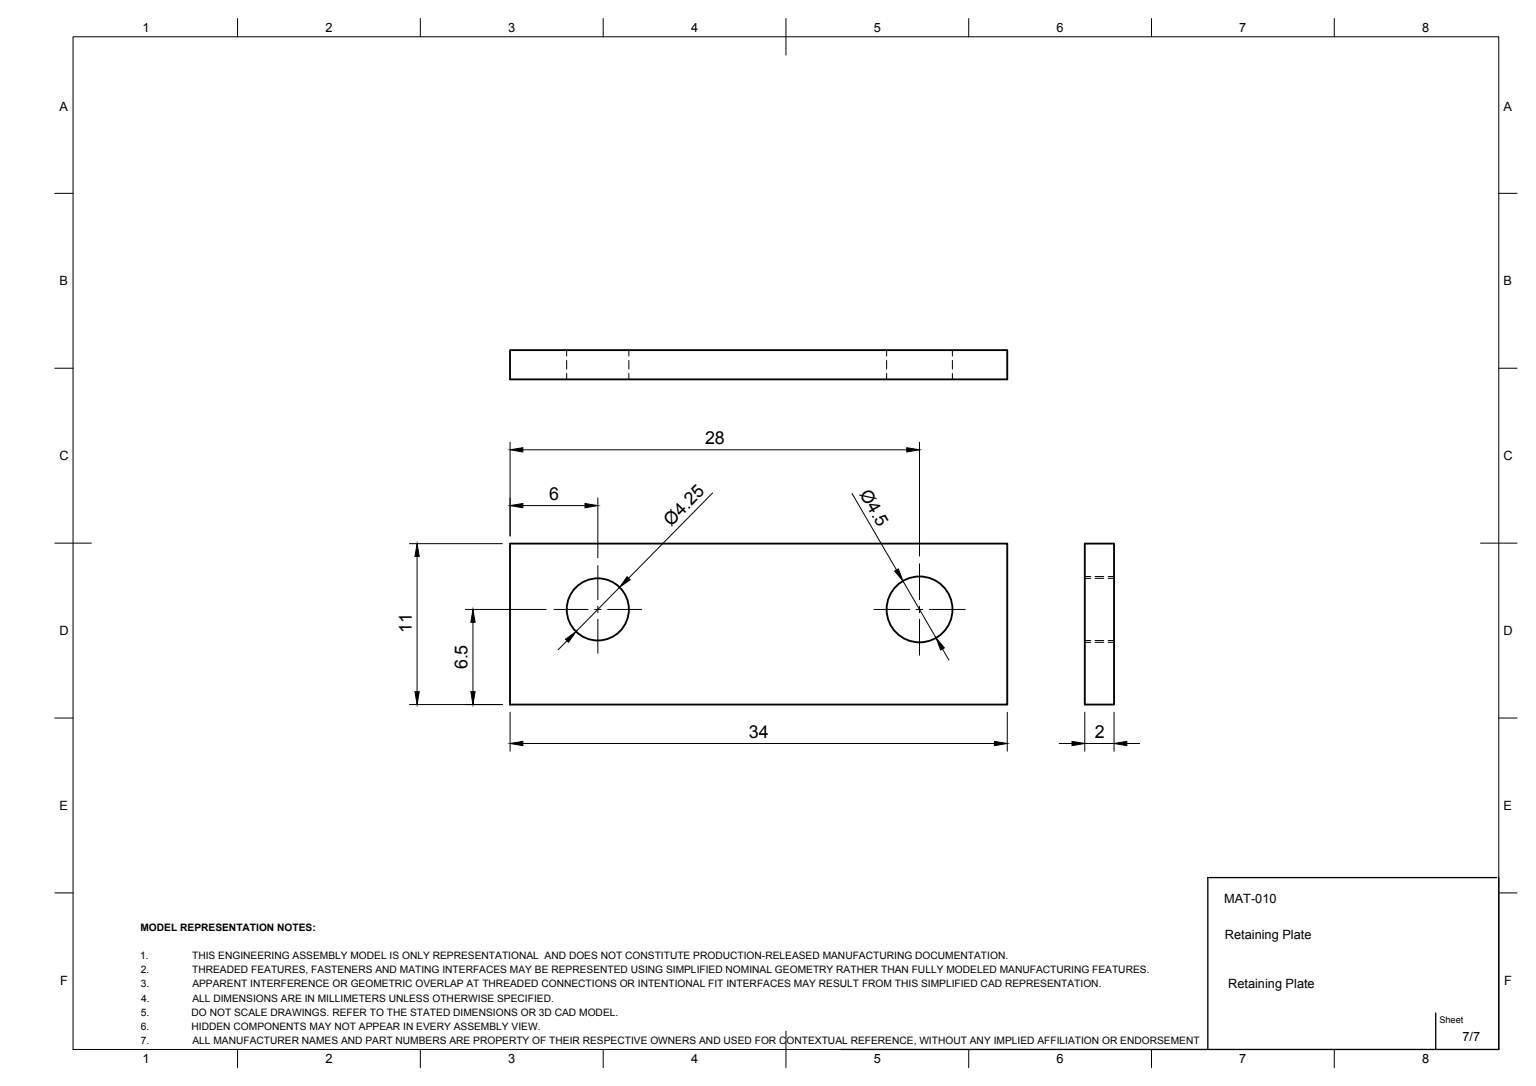
ISO-10303-21;
HEADER;
/* Generated by software containing ST-Developer
 * from STEP Tools, Inc. (www.steptools.com) 
 */

FILE_DESCRIPTION(
/* description */ ('STEP AP214'),
/* implementation_level */ '2;1');

FILE_NAME(
/* name */ 'Retaining Plate.step',
/* time_stamp */ '2026-11-14T05:50:49-08:00',
/* author */ (''),
/* organization */ (''),
/* preprocessor_version */ 'ST-DEVELOPER v20.2',
/* originating_system */ 'Autodesk Translation Framework v15.17.0.0',
/* authorisation */ '');

FILE_SCHEMA (('AUTOMOTIVE_DESIGN { 1 0 10303 214 3 1 1 }'));
ENDSEC;

DATA;
#10=MECHANICAL_DESIGN_GEOMETRIC_PRESENTATION_REPRESENTATION('',(#162),#9903);
#148=SHAPE_REPRESENTATION_RELATIONSHIP('SRR','None',#9943,#155);
#155=ADVANCED_BREP_SHAPE_REPRESENTATION('',(#169),#9901);
#162=STYLED_ITEM('',(#9984),#169);
#169=MANIFOLD_SOLID_BREP('Body1',#2027);
#191=FACE_BOUND('',#446,.T.);
#192=FACE_BOUND('',#447,.T.);
#193=FACE_BOUND('',#449,.T.);
#194=FACE_BOUND('',#450,.T.);
#224=PLANE('',#2228);
#225=PLANE('',#2229);
#226=PLANE('',#2230);
#227=PLANE('',#2231);
#228=PLANE('',#2232);
#229=PLANE('',#2233);
#305=FACE_OUTER_BOUND('',#443,.T.);
#306=FACE_OUTER_BOUND('',#444,.T.);
#307=FACE_OUTER_BOUND('',#445,.T.);
#308=FACE_OUTER_BOUND('',#448,.T.);
#309=FACE_OUTER_BOUND('',#451,.T.);
#310=FACE_OUTER_BOUND('',#452,.T.);
#311=FACE_OUTER_BOUND('',#453,.T.);
#312=FACE_OUTER_BOUND('',#454,.T.);
#443=EDGE_LOOP('',(#1520,#1521,#1522,#1523));
#444=EDGE_LOOP('',(#1524,#1525,#1526,#1527));
#445=EDGE_LOOP('',(#1528,#1529,#1530,#1531));
#446=EDGE_LOOP('',(#1532));
#447=EDGE_LOOP('',(#1533));
#448=EDGE_LOOP('',(#1534,#1535,#1536,#1537));
#449=EDGE_LOOP('',(#1538));
#450=EDGE_LOOP('',(#1539));
#451=EDGE_LOOP('',(#1540,#1541,#1542,#1543));
#452=EDGE_LOOP('',(#1544,#1545,#1546,#1547));
#453=EDGE_LOOP('',(#1548,#1549,#1550,#1551));
#454=EDGE_LOOP('',(#1552,#1553,#1554,#1555));
#563=LINE('',#3113,#699);
#564=LINE('',#3119,#700);
#565=LINE('',#3124,#701);
#566=LINE('',#3126,#702);
#567=LINE('',#3128,#703);
#568=LINE('',#3129,#704);
#569=LINE('',#3133,#705);
#570=LINE('',#3135,#706);
#571=LINE('',#3137,#707);
#572=LINE('',#3138,#708);
#573=LINE('',#3140,#709);
#574=LINE('',#3141,#710);
#575=LINE('',#3143,#711);
#576=LINE('',#3145,#712);
#699=VECTOR('',#2602,2.125);
#700=VECTOR('',#2609,2.25);
#701=VECTOR('',#2614,1000.);
#702=VECTOR('',#2615,1000.);
#703=VECTOR('',#2616,1000.);
#704=VECTOR('',#2617,1000.);
#705=VECTOR('',#2620,1000.);
#706=VECTOR('',#2621,1000.);
#707=VECTOR('',#2622,1000.);
#708=VECTOR('',#2623,1000.);
#709=VECTOR('',#2626,1000.);
#710=VECTOR('',#2627,1000.);
#711=VECTOR('',#2630,1000.);
#712=VECTOR('',#2633,1000.);
#840=CIRCLE('',#2223,2.125);
#841=CIRCLE('',#2224,2.125);
#842=CIRCLE('',#2226,2.25);
#843=CIRCLE('',#2227,2.25);
#927=VERTEX_POINT('',#3110);
#928=VERTEX_POINT('',#3112);
#929=VERTEX_POINT('',#3116);
#930=VERTEX_POINT('',#3118);
#931=VERTEX_POINT('',#3122);
#932=VERTEX_POINT('',#3123);
#933=VERTEX_POINT('',#3125);
#934=VERTEX_POINT('',#3127);
#935=VERTEX_POINT('',#3131);
#936=VERTEX_POINT('',#3132);
#937=VERTEX_POINT('',#3134);
#938=VERTEX_POINT('',#3136);
#1141=EDGE_CURVE('',#927,#927,#840,.T.);
#1142=EDGE_CURVE('',#927,#928,#563,.T.);
#1143=EDGE_CURVE('',#928,#928,#841,.T.);
#1144=EDGE_CURVE('',#929,#929,#842,.T.);
#1145=EDGE_CURVE('',#929,#930,#564,.T.);
#1146=EDGE_CURVE('',#930,#930,#843,.T.);
#1147=EDGE_CURVE('',#931,#932,#565,.T.);
#1148=EDGE_CURVE('',#932,#933,#566,.T.);
#1149=EDGE_CURVE('',#933,#934,#567,.T.);
#1150=EDGE_CURVE('',#934,#931,#568,.T.);
#1151=EDGE_CURVE('',#935,#936,#569,.T.);
#1152=EDGE_CURVE('',#937,#935,#570,.T.);
#1153=EDGE_CURVE('',#938,#937,#571,.T.);
#1154=EDGE_CURVE('',#936,#938,#572,.T.);
#1155=EDGE_CURVE('',#932,#936,#573,.T.);
#1156=EDGE_CURVE('',#931,#935,#574,.T.);
#1157=EDGE_CURVE('',#933,#938,#575,.T.);
#1158=EDGE_CURVE('',#934,#937,#576,.T.);
#1520=ORIENTED_EDGE('',*,*,#1141,.T.);
#1521=ORIENTED_EDGE('',*,*,#1142,.T.);
#1522=ORIENTED_EDGE('',*,*,#1143,.F.);
#1523=ORIENTED_EDGE('',*,*,#1142,.F.);
#1524=ORIENTED_EDGE('',*,*,#1144,.T.);
#1525=ORIENTED_EDGE('',*,*,#1145,.T.);
#1526=ORIENTED_EDGE('',*,*,#1146,.F.);
#1527=ORIENTED_EDGE('',*,*,#1145,.F.);
#1528=ORIENTED_EDGE('',*,*,#1147,.T.);
#1529=ORIENTED_EDGE('',*,*,#1148,.T.);
#1530=ORIENTED_EDGE('',*,*,#1149,.T.);
#1531=ORIENTED_EDGE('',*,*,#1150,.T.);
#1532=ORIENTED_EDGE('',*,*,#1141,.F.);
#1533=ORIENTED_EDGE('',*,*,#1144,.F.);
#1534=ORIENTED_EDGE('',*,*,#1151,.F.);
#1535=ORIENTED_EDGE('',*,*,#1152,.F.);
#1536=ORIENTED_EDGE('',*,*,#1153,.F.);
#1537=ORIENTED_EDGE('',*,*,#1154,.F.);
#1538=ORIENTED_EDGE('',*,*,#1143,.T.);
#1539=ORIENTED_EDGE('',*,*,#1146,.T.);
#1540=ORIENTED_EDGE('',*,*,#1151,.T.);
#1541=ORIENTED_EDGE('',*,*,#1155,.F.);
#1542=ORIENTED_EDGE('',*,*,#1147,.F.);
#1543=ORIENTED_EDGE('',*,*,#1156,.T.);
#1544=ORIENTED_EDGE('',*,*,#1154,.T.);
#1545=ORIENTED_EDGE('',*,*,#1157,.F.);
#1546=ORIENTED_EDGE('',*,*,#1148,.F.);
#1547=ORIENTED_EDGE('',*,*,#1155,.T.);
#1548=ORIENTED_EDGE('',*,*,#1153,.T.);
#1549=ORIENTED_EDGE('',*,*,#1158,.F.);
#1550=ORIENTED_EDGE('',*,*,#1149,.F.);
#1551=ORIENTED_EDGE('',*,*,#1157,.T.);
#1552=ORIENTED_EDGE('',*,*,#1152,.T.);
#1553=ORIENTED_EDGE('',*,*,#1156,.F.);
#1554=ORIENTED_EDGE('',*,*,#1150,.F.);
#1555=ORIENTED_EDGE('',*,*,#1158,.T.);
#1874=CYLINDRICAL_SURFACE('',#2222,2.125);
#1875=CYLINDRICAL_SURFACE('',#2225,2.25);
#1957=ADVANCED_FACE('',(#305),#1874,.F.);
#1958=ADVANCED_FACE('',(#306),#1875,.F.);
#1959=ADVANCED_FACE('',(#307,#191,#192),#224,.T.);
#1960=ADVANCED_FACE('',(#308,#193,#194),#225,.F.);
#1961=ADVANCED_FACE('',(#309),#226,.F.);
#1962=ADVANCED_FACE('',(#310),#227,.F.);
#1963=ADVANCED_FACE('',(#311),#228,.F.);
#1964=ADVANCED_FACE('',(#312),#229,.F.);
#2027=CLOSED_SHELL('',(#1957,#1958,#1959,#1960,#1961,#1962,#1963,#1964));
#2221=AXIS2_PLACEMENT_3D('',#3108,#2596,#2597);
#2222=AXIS2_PLACEMENT_3D('',#3109,#2598,#2599);
#2223=AXIS2_PLACEMENT_3D('',#3111,#2600,#2601);
#2224=AXIS2_PLACEMENT_3D('',#3114,#2603,#2604);
#2225=AXIS2_PLACEMENT_3D('',#3115,#2605,#2606);
#2226=AXIS2_PLACEMENT_3D('',#3117,#2607,#2608);
#2227=AXIS2_PLACEMENT_3D('',#3120,#2610,#2611);
#2228=AXIS2_PLACEMENT_3D('',#3121,#2612,#2613);
#2229=AXIS2_PLACEMENT_3D('',#3130,#2618,#2619);
#2230=AXIS2_PLACEMENT_3D('',#3139,#2624,#2625);
#2231=AXIS2_PLACEMENT_3D('',#3142,#2628,#2629);
#2232=AXIS2_PLACEMENT_3D('',#3144,#2631,#2632);
#2233=AXIS2_PLACEMENT_3D('',#3146,#2634,#2635);
#2596=DIRECTION('axis',(0.,0.,1.));
#2597=DIRECTION('refdir',(1.,0.,0.));
#2598=DIRECTION('center_axis',(0.,0.,-1.));
#2599=DIRECTION('ref_axis',(-1.,0.,0.));
#2600=DIRECTION('center_axis',(0.,0.,1.));
#2601=DIRECTION('ref_axis',(1.,0.,0.));
#2602=DIRECTION('',(0.,0.,-1.));
#2603=DIRECTION('center_axis',(0.,0.,1.));
#2604=DIRECTION('ref_axis',(1.,0.,0.));
#2605=DIRECTION('center_axis',(0.,0.,-1.));
#2606=DIRECTION('ref_axis',(-1.,0.,0.));
#2607=DIRECTION('center_axis',(0.,0.,1.));
#2608=DIRECTION('ref_axis',(1.,0.,0.));
#2609=DIRECTION('',(0.,0.,-1.));
#2610=DIRECTION('center_axis',(0.,0.,1.));
#2611=DIRECTION('ref_axis',(1.,0.,0.));
#2612=DIRECTION('center_axis',(0.,0.,1.));
#2613=DIRECTION('ref_axis',(1.,0.,0.));
#2614=DIRECTION('',(0.,-1.,0.));
#2615=DIRECTION('',(1.,0.,0.));
#2616=DIRECTION('',(0.,1.,0.));
#2617=DIRECTION('',(-1.,0.,0.));
#2618=DIRECTION('center_axis',(0.,0.,1.));
#2619=DIRECTION('ref_axis',(1.,0.,0.));
#2620=DIRECTION('',(0.,-1.,0.));
#2621=DIRECTION('',(-1.,0.,0.));
#2622=DIRECTION('',(0.,1.,0.));
#2623=DIRECTION('',(1.,0.,0.));
#2624=DIRECTION('center_axis',(1.,0.,0.));
#2625=DIRECTION('ref_axis',(0.,0.,-1.));
#2626=DIRECTION('',(0.,0.,-1.));
#2627=DIRECTION('',(0.,0.,-1.));
#2628=DIRECTION('center_axis',(0.,1.,0.));
#2629=DIRECTION('ref_axis',(0.,0.,1.));
#2630=DIRECTION('',(0.,0.,-1.));
#2631=DIRECTION('center_axis',(-1.,0.,0.));
#2632=DIRECTION('ref_axis',(0.,0.,1.));
#2633=DIRECTION('',(0.,0.,-1.));
#2634=DIRECTION('center_axis',(0.,-1.,0.));
#2635=DIRECTION('ref_axis',(0.,0.,-1.));
#3108=CARTESIAN_POINT('',(0.,0.,0.));
#3109=CARTESIAN_POINT('Origin',(28.,6.5,2.));
#3110=CARTESIAN_POINT('',(30.125,6.5,2.));
#3111=CARTESIAN_POINT('Origin',(28.,6.5,2.));
#3112=CARTESIAN_POINT('',(30.125,6.5,0.));
#3113=CARTESIAN_POINT('',(30.125,6.5,2.));
#3114=CARTESIAN_POINT('Origin',(28.,6.5,0.));
#3115=CARTESIAN_POINT('Origin',(6.,6.5,2.));
#3116=CARTESIAN_POINT('',(8.25,6.5,2.));
#3117=CARTESIAN_POINT('Origin',(6.,6.5,2.));
#3118=CARTESIAN_POINT('',(8.25,6.5,0.));
#3119=CARTESIAN_POINT('',(8.25,6.5,2.));
#3120=CARTESIAN_POINT('Origin',(6.,6.5,0.));
#3121=CARTESIAN_POINT('Origin',(0.,0.,2.));
#3122=CARTESIAN_POINT('',(0.,11.,2.));
#3123=CARTESIAN_POINT('',(0.,0.,2.));
#3124=CARTESIAN_POINT('',(0.,11.,2.));
#3125=CARTESIAN_POINT('',(34.,0.,2.));
#3126=CARTESIAN_POINT('',(0.,0.,2.));
#3127=CARTESIAN_POINT('',(34.,11.,2.));
#3128=CARTESIAN_POINT('',(34.,0.,2.));
#3129=CARTESIAN_POINT('',(34.,11.,2.));
#3130=CARTESIAN_POINT('Origin',(0.,0.,0.));
#3131=CARTESIAN_POINT('',(0.,11.,0.));
#3132=CARTESIAN_POINT('',(0.,0.,0.));
#3133=CARTESIAN_POINT('',(0.,11.,0.));
#3134=CARTESIAN_POINT('',(34.,11.,0.));
#3135=CARTESIAN_POINT('',(34.,11.,0.));
#3136=CARTESIAN_POINT('',(34.,0.,0.));
#3137=CARTESIAN_POINT('',(34.,0.,0.));
#3138=CARTESIAN_POINT('',(0.,0.,0.));
#3139=CARTESIAN_POINT('Origin',(0.,11.,2.));
#3140=CARTESIAN_POINT('',(0.,0.,2.));
#3141=CARTESIAN_POINT('',(0.,11.,2.));
#3142=CARTESIAN_POINT('Origin',(0.,0.,2.));
#3143=CARTESIAN_POINT('',(34.,0.,2.));
#3144=CARTESIAN_POINT('Origin',(34.,0.,2.));
#3145=CARTESIAN_POINT('',(34.,11.,2.));
#3146=CARTESIAN_POINT('Origin',(34.,11.,2.));
#9892=UNCERTAINTY_MEASURE_WITH_UNIT(LENGTH_MEASURE(0.01),#9904,
'DISTANCE_ACCURACY_VALUE',
'Maximum model space distance between geometric entities at asserted c
onnectivities');
#9894=UNCERTAINTY_MEASURE_WITH_UNIT(LENGTH_MEASURE(0.01),#9904,
'DISTANCE_ACCURACY_VALUE',
'Maximum model space distance between geometric entities at asserted c
onnectivities');
#9901=(
GEOMETRIC_REPRESENTATION_CONTEXT(3)
GLOBAL_UNCERTAINTY_ASSIGNED_CONTEXT((#9892))
GLOBAL_UNIT_ASSIGNED_CONTEXT((#9904,#9906,#9907))
REPRESENTATION_CONTEXT('','3D')
);
#9903=(
GEOMETRIC_REPRESENTATION_CONTEXT(3)
GLOBAL_UNCERTAINTY_ASSIGNED_CONTEXT((#9894))
GLOBAL_UNIT_ASSIGNED_CONTEXT((#9904,#9906,#9907))
REPRESENTATION_CONTEXT('','3D')
);
#9904=(
LENGTH_UNIT()
NAMED_UNIT(*)
SI_UNIT(.MILLI.,.METRE.)
);
#9906=(
NAMED_UNIT(*)
PLANE_ANGLE_UNIT()
SI_UNIT($,.RADIAN.)
);
#9907=(
NAMED_UNIT(*)
SI_UNIT($,.STERADIAN.)
SOLID_ANGLE_UNIT()
);
#9914=SHAPE_DEFINITION_REPRESENTATION(#9922,#9943);
#9922=PRODUCT_DEFINITION_SHAPE('',$,#9952);
#9943=SHAPE_REPRESENTATION('',(#2221),#9901);
#9945=PRODUCT_DEFINITION_CONTEXT('part definition',#9971,'design');
#9952=PRODUCT_DEFINITION('Retaining Plate','Retaining Plate',#9960,#9945);
#9960=PRODUCT_DEFINITION_FORMATION('',$,#9979);
#9971=APPLICATION_CONTEXT(
'Core Data for Automotive Mechanical Design Process');
#9972=PRODUCT_CONTEXT('part definition',#9971,'mechanical');
#9979=PRODUCT('Retaining Plate','Retaining Plate',$,(#9972));
#9984=PRESENTATION_STYLE_ASSIGNMENT((#9989));
#9989=SURFACE_STYLE_USAGE(.BOTH.,#9994);
#9994=SURFACE_SIDE_STYLE('',(#9999));
#9999=SURFACE_STYLE_FILL_AREA(#10004);
#10004=FILL_AREA_STYLE('Opaque(227,224,212)',(#10009));
#10009=FILL_AREA_STYLE_COLOUR('Opaque(227,224,212)',#10014);
#10014=COLOUR_RGB('Opaque(227,224,212)',0.890196078431372,0.87843137254902,
0.831372549019608);
ENDSEC;
END-ISO-10303-21;
